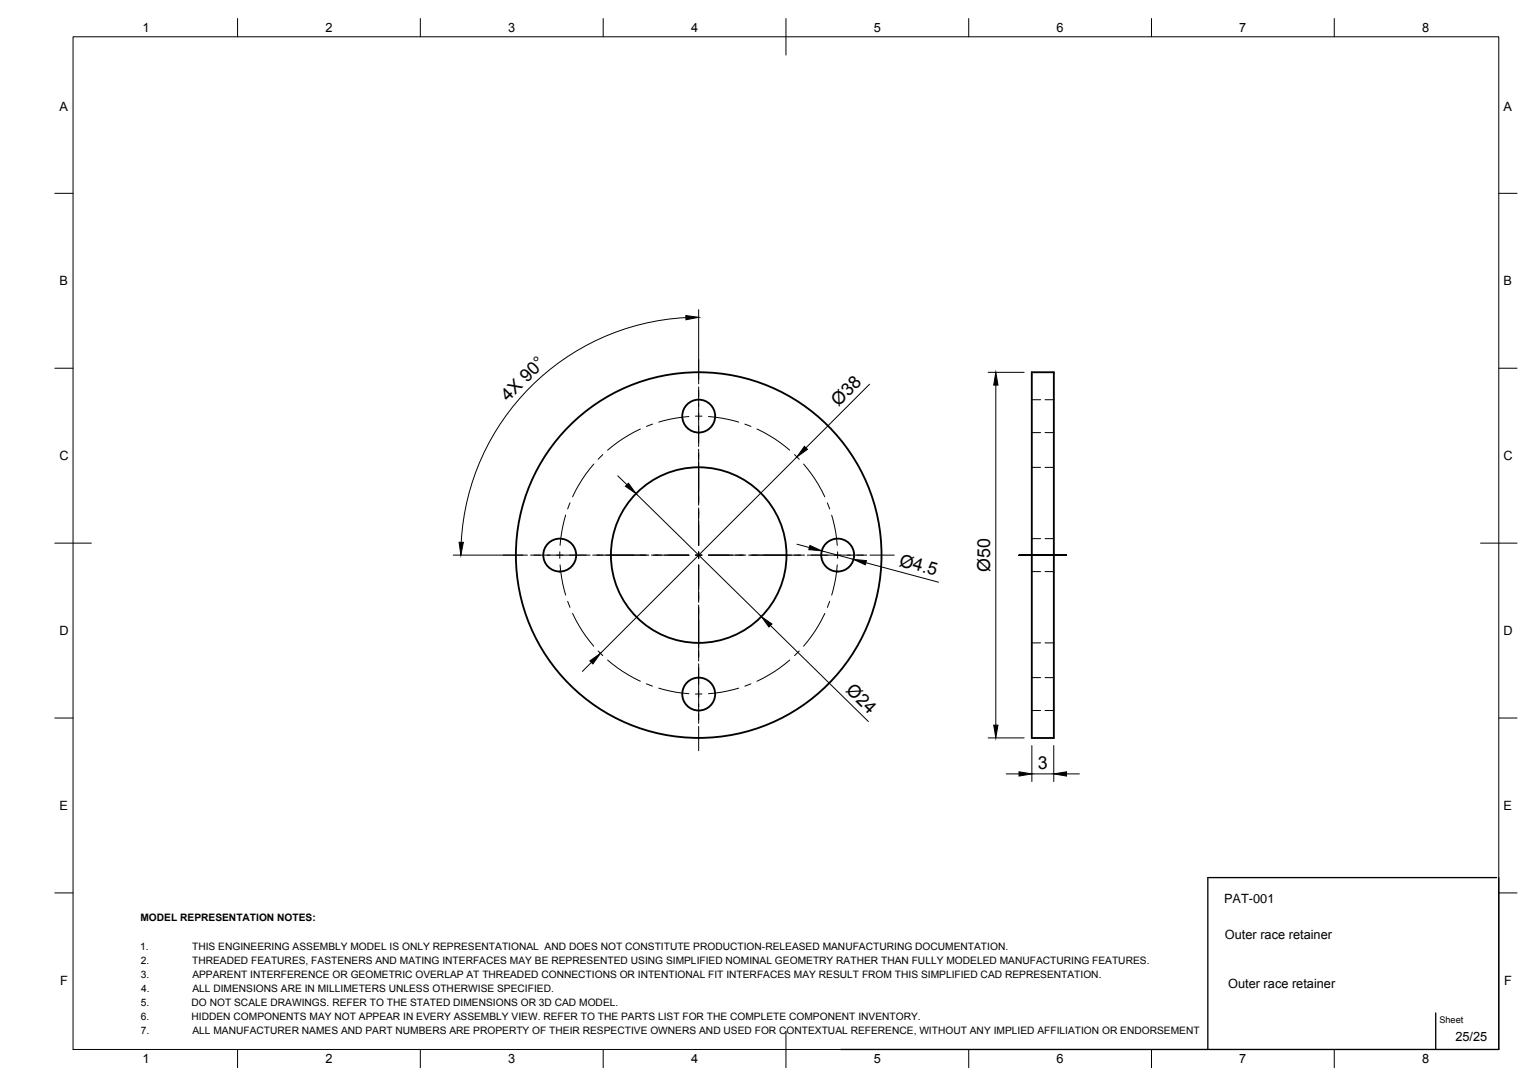
ISO-10303-21;
HEADER;
/* Generated by software containing ST-Developer
 * from STEP Tools, Inc. (www.steptools.com) 
 */

FILE_DESCRIPTION(
/* description */ ('PAT-001'),
/* implementation_level */ '2;1');

FILE_NAME(
/* name */ 'Outer race retainer.step',
/* time_stamp */ '2026-10-29T17:07:15-07:00',
/* author */ (''),
/* organization */ (''),
/* preprocessor_version */ 'ST-DEVELOPER v20.2',
/* originating_system */ 'Autodesk Translation Framework v15.17.0.0',
/* authorisation */ '');

FILE_SCHEMA (('AUTOMOTIVE_DESIGN { 1 0 10303 214 3 1 1 }'));
ENDSEC;

DATA;
#10=MECHANICAL_DESIGN_GEOMETRIC_PRESENTATION_REPRESENTATION('',(#404),#9622);
#346=SHAPE_REPRESENTATION_RELATIONSHIP('SRR','None',#9771,#371);
#371=ADVANCED_BREP_SHAPE_REPRESENTATION('',(#436),#9620);
#404=STYLED_ITEM('',(#9962),#436);
#436=MANIFOLD_SOLID_BREP('Body1',#5230);
#517=FACE_BOUND('',#1369,.T.);
#518=FACE_BOUND('',#1370,.T.);
#519=FACE_BOUND('',#1371,.T.);
#520=FACE_BOUND('',#1372,.T.);
#521=FACE_BOUND('',#1373,.T.);
#522=FACE_BOUND('',#1375,.T.);
#523=FACE_BOUND('',#1376,.T.);
#524=FACE_BOUND('',#1377,.T.);
#525=FACE_BOUND('',#1378,.T.);
#526=FACE_BOUND('',#1379,.T.);
#702=PLANE('',#6025);
#703=PLANE('',#6026);
#986=FACE_OUTER_BOUND('',#1362,.T.);
#987=FACE_OUTER_BOUND('',#1363,.T.);
#988=FACE_OUTER_BOUND('',#1364,.T.);
#989=FACE_OUTER_BOUND('',#1365,.T.);
#990=FACE_OUTER_BOUND('',#1366,.T.);
#991=FACE_OUTER_BOUND('',#1367,.T.);
#992=FACE_OUTER_BOUND('',#1368,.T.);
#993=FACE_OUTER_BOUND('',#1374,.T.);
#1362=EDGE_LOOP('',(#4727,#4728,#4729,#4730));
#1363=EDGE_LOOP('',(#4731,#4732,#4733,#4734));
#1364=EDGE_LOOP('',(#4735,#4736,#4737,#4738));
#1365=EDGE_LOOP('',(#4739,#4740,#4741,#4742));
#1366=EDGE_LOOP('',(#4743,#4744,#4745,#4746));
#1367=EDGE_LOOP('',(#4747,#4748,#4749,#4750));
#1368=EDGE_LOOP('',(#4751));
#1369=EDGE_LOOP('',(#4752));
#1370=EDGE_LOOP('',(#4753));
#1371=EDGE_LOOP('',(#4754));
#1372=EDGE_LOOP('',(#4755));
#1373=EDGE_LOOP('',(#4756));
#1374=EDGE_LOOP('',(#4757));
#1375=EDGE_LOOP('',(#4758));
#1376=EDGE_LOOP('',(#4759));
#1377=EDGE_LOOP('',(#4760));
#1378=EDGE_LOOP('',(#4761));
#1379=EDGE_LOOP('',(#4762));
#1773=LINE('',#9405,#2178);
#1774=LINE('',#9411,#2179);
#1775=LINE('',#9417,#2180);
#1776=LINE('',#9423,#2181);
#1777=LINE('',#9429,#2182);
#1778=LINE('',#9435,#2183);
#2178=VECTOR('',#7482,0.225);
#2179=VECTOR('',#7489,0.225);
#2180=VECTOR('',#7496,0.225);
#2181=VECTOR('',#7503,0.225);
#2182=VECTOR('',#7510,1.2);
#2183=VECTOR('',#7517,2.5);
#2400=CIRCLE('',#6008,0.225);
#2401=CIRCLE('',#6009,0.225);
#2402=CIRCLE('',#6011,0.225);
#2403=CIRCLE('',#6012,0.225);
#2404=CIRCLE('',#6014,0.225);
#2405=CIRCLE('',#6015,0.225);
#2406=CIRCLE('',#6017,0.225);
#2407=CIRCLE('',#6018,0.225);
#2408=CIRCLE('',#6020,1.2);
#2409=CIRCLE('',#6021,1.2);
#2410=CIRCLE('',#6023,2.5);
#2411=CIRCLE('',#6024,2.5);
#2830=VERTEX_POINT('',#9402);
#2831=VERTEX_POINT('',#9404);
#2832=VERTEX_POINT('',#9408);
#2833=VERTEX_POINT('',#9410);
#2834=VERTEX_POINT('',#9414);
#2835=VERTEX_POINT('',#9416);
#2836=VERTEX_POINT('',#9420);
#2837=VERTEX_POINT('',#9422);
#2838=VERTEX_POINT('',#9426);
#2839=VERTEX_POINT('',#9428);
#2840=VERTEX_POINT('',#9432);
#2841=VERTEX_POINT('',#9434);
#3467=EDGE_CURVE('',#2830,#2830,#2400,.T.);
#3468=EDGE_CURVE('',#2830,#2831,#1773,.T.);
#3469=EDGE_CURVE('',#2831,#2831,#2401,.T.);
#3470=EDGE_CURVE('',#2832,#2832,#2402,.T.);
#3471=EDGE_CURVE('',#2832,#2833,#1774,.T.);
#3472=EDGE_CURVE('',#2833,#2833,#2403,.T.);
#3473=EDGE_CURVE('',#2834,#2834,#2404,.T.);
#3474=EDGE_CURVE('',#2834,#2835,#1775,.T.);
#3475=EDGE_CURVE('',#2835,#2835,#2405,.T.);
#3476=EDGE_CURVE('',#2836,#2836,#2406,.T.);
#3477=EDGE_CURVE('',#2836,#2837,#1776,.T.);
#3478=EDGE_CURVE('',#2837,#2837,#2407,.T.);
#3479=EDGE_CURVE('',#2838,#2838,#2408,.T.);
#3480=EDGE_CURVE('',#2838,#2839,#1777,.T.);
#3481=EDGE_CURVE('',#2839,#2839,#2409,.T.);
#3482=EDGE_CURVE('',#2840,#2840,#2410,.T.);
#3483=EDGE_CURVE('',#2840,#2841,#1778,.T.);
#3484=EDGE_CURVE('',#2841,#2841,#2411,.T.);
#4727=ORIENTED_EDGE('',*,*,#3467,.F.);
#4728=ORIENTED_EDGE('',*,*,#3468,.T.);
#4729=ORIENTED_EDGE('',*,*,#3469,.F.);
#4730=ORIENTED_EDGE('',*,*,#3468,.F.);
#4731=ORIENTED_EDGE('',*,*,#3470,.F.);
#4732=ORIENTED_EDGE('',*,*,#3471,.T.);
#4733=ORIENTED_EDGE('',*,*,#3472,.F.);
#4734=ORIENTED_EDGE('',*,*,#3471,.F.);
#4735=ORIENTED_EDGE('',*,*,#3473,.F.);
#4736=ORIENTED_EDGE('',*,*,#3474,.T.);
#4737=ORIENTED_EDGE('',*,*,#3475,.F.);
#4738=ORIENTED_EDGE('',*,*,#3474,.F.);
#4739=ORIENTED_EDGE('',*,*,#3476,.F.);
#4740=ORIENTED_EDGE('',*,*,#3477,.T.);
#4741=ORIENTED_EDGE('',*,*,#3478,.F.);
#4742=ORIENTED_EDGE('',*,*,#3477,.F.);
#4743=ORIENTED_EDGE('',*,*,#3479,.F.);
#4744=ORIENTED_EDGE('',*,*,#3480,.T.);
#4745=ORIENTED_EDGE('',*,*,#3481,.T.);
#4746=ORIENTED_EDGE('',*,*,#3480,.F.);
#4747=ORIENTED_EDGE('',*,*,#3482,.F.);
#4748=ORIENTED_EDGE('',*,*,#3483,.T.);
#4749=ORIENTED_EDGE('',*,*,#3484,.T.);
#4750=ORIENTED_EDGE('',*,*,#3483,.F.);
#4751=ORIENTED_EDGE('',*,*,#3482,.T.);
#4752=ORIENTED_EDGE('',*,*,#3479,.T.);
#4753=ORIENTED_EDGE('',*,*,#3478,.T.);
#4754=ORIENTED_EDGE('',*,*,#3475,.T.);
#4755=ORIENTED_EDGE('',*,*,#3472,.T.);
#4756=ORIENTED_EDGE('',*,*,#3469,.T.);
#4757=ORIENTED_EDGE('',*,*,#3484,.F.);
#4758=ORIENTED_EDGE('',*,*,#3481,.F.);
#4759=ORIENTED_EDGE('',*,*,#3476,.T.);
#4760=ORIENTED_EDGE('',*,*,#3473,.T.);
#4761=ORIENTED_EDGE('',*,*,#3470,.T.);
#4762=ORIENTED_EDGE('',*,*,#3467,.T.);
#4894=CYLINDRICAL_SURFACE('',#6007,0.225);
#4895=CYLINDRICAL_SURFACE('',#6010,0.225);
#4896=CYLINDRICAL_SURFACE('',#6013,0.225);
#4897=CYLINDRICAL_SURFACE('',#6016,0.225);
#4898=CYLINDRICAL_SURFACE('',#6019,1.2);
#4899=CYLINDRICAL_SURFACE('',#6022,2.5);
#5173=ADVANCED_FACE('',(#986),#4894,.F.);
#5174=ADVANCED_FACE('',(#987),#4895,.F.);
#5175=ADVANCED_FACE('',(#988),#4896,.F.);
#5176=ADVANCED_FACE('',(#989),#4897,.F.);
#5177=ADVANCED_FACE('',(#990),#4898,.F.);
#5178=ADVANCED_FACE('',(#991),#4899,.T.);
#5179=ADVANCED_FACE('',(#992,#517,#518,#519,#520,#521),#702,.T.);
#5180=ADVANCED_FACE('',(#993,#522,#523,#524,#525,#526),#703,.F.);
#5230=CLOSED_SHELL('',(#5173,#5174,#5175,#5176,#5177,#5178,#5179,#5180));
#6006=AXIS2_PLACEMENT_3D('',#9400,#7476,#7477);
#6007=AXIS2_PLACEMENT_3D('',#9401,#7478,#7479);
#6008=AXIS2_PLACEMENT_3D('',#9403,#7480,#7481);
#6009=AXIS2_PLACEMENT_3D('',#9406,#7483,#7484);
#6010=AXIS2_PLACEMENT_3D('',#9407,#7485,#7486);
#6011=AXIS2_PLACEMENT_3D('',#9409,#7487,#7488);
#6012=AXIS2_PLACEMENT_3D('',#9412,#7490,#7491);
#6013=AXIS2_PLACEMENT_3D('',#9413,#7492,#7493);
#6014=AXIS2_PLACEMENT_3D('',#9415,#7494,#7495);
#6015=AXIS2_PLACEMENT_3D('',#9418,#7497,#7498);
#6016=AXIS2_PLACEMENT_3D('',#9419,#7499,#7500);
#6017=AXIS2_PLACEMENT_3D('',#9421,#7501,#7502);
#6018=AXIS2_PLACEMENT_3D('',#9424,#7504,#7505);
#6019=AXIS2_PLACEMENT_3D('',#9425,#7506,#7507);
#6020=AXIS2_PLACEMENT_3D('',#9427,#7508,#7509);
#6021=AXIS2_PLACEMENT_3D('',#9430,#7511,#7512);
#6022=AXIS2_PLACEMENT_3D('',#9431,#7513,#7514);
#6023=AXIS2_PLACEMENT_3D('',#9433,#7515,#7516);
#6024=AXIS2_PLACEMENT_3D('',#9436,#7518,#7519);
#6025=AXIS2_PLACEMENT_3D('',#9437,#7520,#7521);
#6026=AXIS2_PLACEMENT_3D('',#9438,#7522,#7523);
#7476=DIRECTION('axis',(0.,0.,1.));
#7477=DIRECTION('refdir',(1.,0.,0.));
#7478=DIRECTION('center_axis',(0.,1.,0.));
#7479=DIRECTION('ref_axis',(1.,0.,0.));
#7480=DIRECTION('center_axis',(0.,1.,0.));
#7481=DIRECTION('ref_axis',(1.,0.,0.));
#7482=DIRECTION('',(0.,1.,0.));
#7483=DIRECTION('center_axis',(0.,-1.,0.));
#7484=DIRECTION('ref_axis',(1.,0.,0.));
#7485=DIRECTION('center_axis',(0.,1.,0.));
#7486=DIRECTION('ref_axis',(1.,0.,0.));
#7487=DIRECTION('center_axis',(0.,1.,0.));
#7488=DIRECTION('ref_axis',(1.,0.,0.));
#7489=DIRECTION('',(0.,1.,0.));
#7490=DIRECTION('center_axis',(0.,-1.,0.));
#7491=DIRECTION('ref_axis',(1.,0.,0.));
#7492=DIRECTION('center_axis',(0.,1.,0.));
#7493=DIRECTION('ref_axis',(1.,0.,0.));
#7494=DIRECTION('center_axis',(0.,1.,0.));
#7495=DIRECTION('ref_axis',(1.,0.,0.));
#7496=DIRECTION('',(0.,1.,0.));
#7497=DIRECTION('center_axis',(0.,-1.,0.));
#7498=DIRECTION('ref_axis',(1.,0.,0.));
#7499=DIRECTION('center_axis',(0.,1.,0.));
#7500=DIRECTION('ref_axis',(1.,0.,0.));
#7501=DIRECTION('center_axis',(0.,1.,0.));
#7502=DIRECTION('ref_axis',(1.,0.,0.));
#7503=DIRECTION('',(0.,1.,0.));
#7504=DIRECTION('center_axis',(0.,-1.,0.));
#7505=DIRECTION('ref_axis',(1.,0.,0.));
#7506=DIRECTION('center_axis',(0.,1.,0.));
#7507=DIRECTION('ref_axis',(1.,0.,0.));
#7508=DIRECTION('center_axis',(0.,-1.,0.));
#7509=DIRECTION('ref_axis',(1.,0.,0.));
#7510=DIRECTION('',(0.,-1.,0.));
#7511=DIRECTION('center_axis',(0.,-1.,0.));
#7512=DIRECTION('ref_axis',(1.,0.,0.));
#7513=DIRECTION('center_axis',(0.,1.,0.));
#7514=DIRECTION('ref_axis',(1.,0.,0.));
#7515=DIRECTION('center_axis',(0.,1.,0.));
#7516=DIRECTION('ref_axis',(1.,0.,0.));
#7517=DIRECTION('',(0.,-1.,0.));
#7518=DIRECTION('center_axis',(0.,1.,0.));
#7519=DIRECTION('ref_axis',(1.,0.,0.));
#7520=DIRECTION('center_axis',(0.,1.,0.));
#7521=DIRECTION('ref_axis',(1.,0.,0.));
#7522=DIRECTION('center_axis',(0.,1.,0.));
#7523=DIRECTION('ref_axis',(1.,0.,0.));
#9400=CARTESIAN_POINT('',(0.,0.,0.));
#9401=CARTESIAN_POINT('Origin',(-1.9,-0.4,4.5));
#9402=CARTESIAN_POINT('',(-2.125,-0.3,4.5));
#9403=CARTESIAN_POINT('Origin',(-1.9,-0.3,4.5));
#9404=CARTESIAN_POINT('',(-2.125,0.,4.5));
#9405=CARTESIAN_POINT('',(-2.125,-0.4,4.5));
#9406=CARTESIAN_POINT('Origin',(-1.9,0.,4.5));
#9407=CARTESIAN_POINT('Origin',(1.16341445918999E-16,-0.4,6.4));
#9408=CARTESIAN_POINT('',(-0.225,-0.3,6.4));
#9409=CARTESIAN_POINT('Origin',(1.16341445918999E-16,-0.3,6.4));
#9410=CARTESIAN_POINT('',(-0.225,0.,6.4));
#9411=CARTESIAN_POINT('',(-0.225,-0.4,6.4));
#9412=CARTESIAN_POINT('Origin',(1.16341445918999E-16,0.,6.4));
#9413=CARTESIAN_POINT('Origin',(1.9,-0.4,4.5));
#9414=CARTESIAN_POINT('',(1.675,-0.3,4.5));
#9415=CARTESIAN_POINT('Origin',(1.9,-0.3,4.5));
#9416=CARTESIAN_POINT('',(1.675,0.,4.5));
#9417=CARTESIAN_POINT('',(1.675,-0.4,4.5));
#9418=CARTESIAN_POINT('Origin',(1.9,0.,4.5));
#9419=CARTESIAN_POINT('Origin',(-3.49024337756996E-16,-0.4,2.6));
#9420=CARTESIAN_POINT('',(-0.225,-0.3,2.6));
#9421=CARTESIAN_POINT('Origin',(-3.49024337756996E-16,-0.3,2.6));
#9422=CARTESIAN_POINT('',(-0.225,0.,2.6));
#9423=CARTESIAN_POINT('',(-0.225,-0.4,2.6));
#9424=CARTESIAN_POINT('Origin',(-3.49024337756996E-16,0.,2.6));
#9425=CARTESIAN_POINT('Origin',(0.,-0.3,4.5));
#9426=CARTESIAN_POINT('',(-1.2,0.,4.5));
#9427=CARTESIAN_POINT('Origin',(0.,0.,4.5));
#9428=CARTESIAN_POINT('',(-1.2,-0.3,4.5));
#9429=CARTESIAN_POINT('',(-1.2,-0.3,4.5));
#9430=CARTESIAN_POINT('Origin',(0.,-0.3,4.5));
#9431=CARTESIAN_POINT('Origin',(0.,-0.3,4.5));
#9432=CARTESIAN_POINT('',(-2.5,0.,4.5));
#9433=CARTESIAN_POINT('Origin',(0.,0.,4.5));
#9434=CARTESIAN_POINT('',(-2.5,-0.3,4.5));
#9435=CARTESIAN_POINT('',(-2.5,-0.3,4.5));
#9436=CARTESIAN_POINT('Origin',(0.,-0.3,4.5));
#9437=CARTESIAN_POINT('Origin',(0.,0.,4.5));
#9438=CARTESIAN_POINT('Origin',(0.,-0.3,4.5));
#9590=UNCERTAINTY_MEASURE_WITH_UNIT(LENGTH_MEASURE(0.001),#9623,
'DISTANCE_ACCURACY_VALUE',
'Maximum model space distance between geometric entities at asserted c
onnectivities');
#9592=UNCERTAINTY_MEASURE_WITH_UNIT(LENGTH_MEASURE(0.001),#9623,
'DISTANCE_ACCURACY_VALUE',
'Maximum model space distance between geometric entities at asserted c
onnectivities');
#9620=(
GEOMETRIC_REPRESENTATION_CONTEXT(3)
GLOBAL_UNCERTAINTY_ASSIGNED_CONTEXT((#9590))
GLOBAL_UNIT_ASSIGNED_CONTEXT((#9623,#9625,#9626))
REPRESENTATION_CONTEXT('','3D')
);
#9622=(
GEOMETRIC_REPRESENTATION_CONTEXT(3)
GLOBAL_UNCERTAINTY_ASSIGNED_CONTEXT((#9592))
GLOBAL_UNIT_ASSIGNED_CONTEXT((#9623,#9625,#9626))
REPRESENTATION_CONTEXT('','3D')
);
#9623=(
LENGTH_UNIT()
NAMED_UNIT(*)
SI_UNIT(.CENTI.,.METRE.)
);
#9625=(
NAMED_UNIT(*)
PLANE_ANGLE_UNIT()
SI_UNIT($,.RADIAN.)
);
#9626=(
NAMED_UNIT(*)
SI_UNIT($,.STERADIAN.)
SOLID_ANGLE_UNIT()
);
#9654=SHAPE_DEFINITION_REPRESENTATION(#9688,#9771);
#9688=PRODUCT_DEFINITION_SHAPE('',$,#9801);
#9771=SHAPE_REPRESENTATION('',(#6006),#9620);
#9773=PRODUCT_DEFINITION_CONTEXT('part definition',#9862,'design');
#9801=PRODUCT_DEFINITION('Outer race retainer','Outer race retainer',#9830,
#9773);
#9830=PRODUCT_DEFINITION_FORMATION('',$,#9891);
#9862=APPLICATION_CONTEXT(
'Core Data for Automotive Mechanical Design Process');
#9863=PRODUCT_CONTEXT('part definition',#9862,'mechanical');
#9891=PRODUCT('Outer race retainer','Outer race retainer',
'Outer race retainer',(#9863));
#9956=COLOUR_RGB('Grey',0.48,0.52,0.57);
#9957=FILL_AREA_STYLE_COLOUR('',#9956);
#9958=FILL_AREA_STYLE('',(#9957));
#9959=SURFACE_STYLE_FILL_AREA(#9958);
#9960=SURFACE_SIDE_STYLE('',(#9959));
#9961=SURFACE_STYLE_USAGE(.BOTH.,#9960);
#9962=PRESENTATION_STYLE_ASSIGNMENT((#9961));
ENDSEC;
END-ISO-10303-21;
